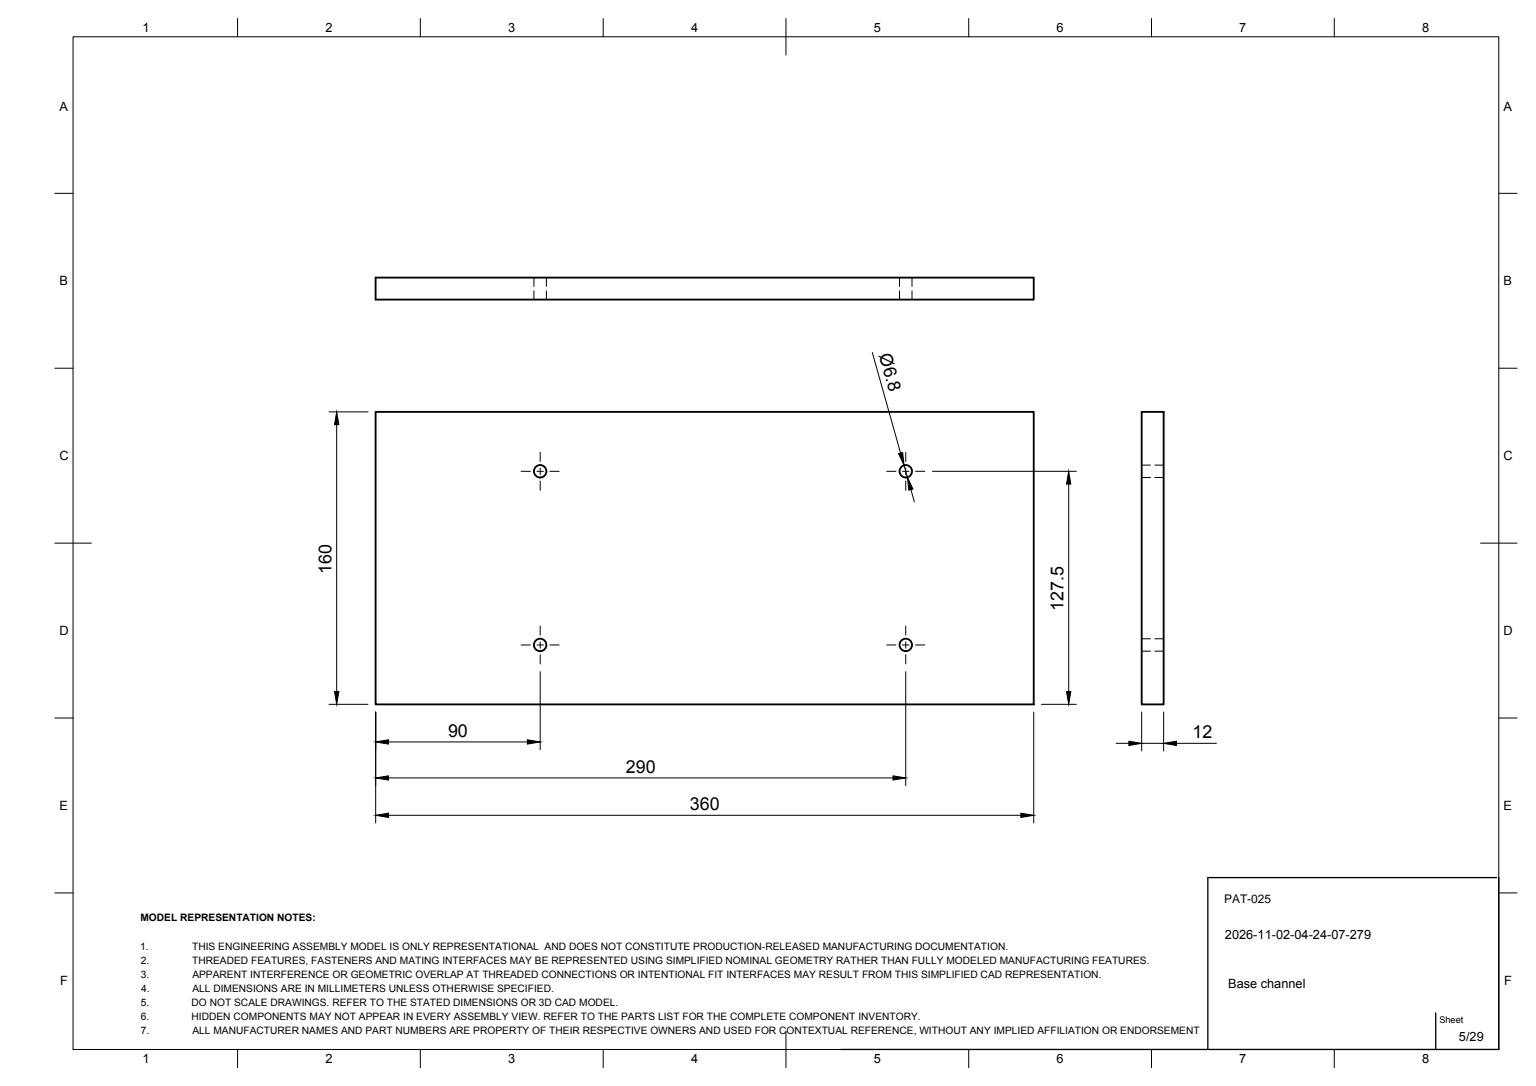
ISO-10303-21;
HEADER;
/* Generated by software containing ST-Developer
 * from STEP Tools, Inc. (www.steptools.com) 
 */

FILE_DESCRIPTION(
/* description */ ('Counter shaft with two pulleys and keyed hub'),
/* implementation_level */ '2;1');

FILE_NAME(
/* name */ 'Base channel.step',
/* time_stamp */ '2026-10-27T10:46:10-07:00',
/* author */ (''),
/* organization */ (''),
/* preprocessor_version */ 'ST-DEVELOPER v20.2',
/* originating_system */ 'Autodesk Translation Framework v15.17.0.0',
/* authorisation */ '');

FILE_SCHEMA (('AUTOMOTIVE_DESIGN { 1 0 10303 214 3 1 1 }'));
ENDSEC;

DATA;
#10=MECHANICAL_DESIGN_GEOMETRIC_PRESENTATION_REPRESENTATION('',(#290),#10821);
#240=SHAPE_REPRESENTATION_RELATIONSHIP('SRR','None',#10926,#265);
#265=ADVANCED_BREP_SHAPE_REPRESENTATION('',(#316),#10794);
#290=STYLED_ITEM('',(#11114),#316);
#316=MANIFOLD_SOLID_BREP('Body1',#5573);
#340=FACE_BOUND('',#911,.T.);
#341=FACE_BOUND('',#912,.T.);
#342=FACE_BOUND('',#913,.T.);
#343=FACE_BOUND('',#914,.T.);
#344=FACE_BOUND('',#916,.T.);
#345=FACE_BOUND('',#917,.T.);
#346=FACE_BOUND('',#918,.T.);
#347=FACE_BOUND('',#919,.T.);
#431=PLANE('',#5892);
#432=PLANE('',#5893);
#433=PLANE('',#5894);
#434=PLANE('',#5895);
#435=PLANE('',#5896);
#436=PLANE('',#5897);
#588=FACE_OUTER_BOUND('',#902,.T.);
#589=FACE_OUTER_BOUND('',#903,.T.);
#590=FACE_OUTER_BOUND('',#904,.T.);
#591=FACE_OUTER_BOUND('',#905,.T.);
#592=FACE_OUTER_BOUND('',#906,.T.);
#593=FACE_OUTER_BOUND('',#907,.T.);
#594=FACE_OUTER_BOUND('',#908,.T.);
#595=FACE_OUTER_BOUND('',#909,.T.);
#596=FACE_OUTER_BOUND('',#910,.T.);
#597=FACE_OUTER_BOUND('',#915,.T.);
#902=EDGE_LOOP('',(#3629,#3630,#3631,#3632));
#903=EDGE_LOOP('',(#3633,#3634,#3635,#3636));
#904=EDGE_LOOP('',(#3637,#3638,#3639,#3640));
#905=EDGE_LOOP('',(#3641,#3642,#3643,#3644));
#906=EDGE_LOOP('',(#3645,#3646,#3647,#3648));
#907=EDGE_LOOP('',(#3649,#3650,#3651,#3652));
#908=EDGE_LOOP('',(#3653,#3654,#3655,#3656));
#909=EDGE_LOOP('',(#3657,#3658,#3659,#3660));
#910=EDGE_LOOP('',(#3661,#3662,#3663,#3664));
#911=EDGE_LOOP('',(#3665));
#912=EDGE_LOOP('',(#3666));
#913=EDGE_LOOP('',(#3667));
#914=EDGE_LOOP('',(#3668));
#915=EDGE_LOOP('',(#3669,#3670,#3671,#3672));
#916=EDGE_LOOP('',(#3673));
#917=EDGE_LOOP('',(#3674));
#918=EDGE_LOOP('',(#3675));
#919=EDGE_LOOP('',(#3676));
#1307=LINE('',#8319,#1696);
#1308=LINE('',#8325,#1697);
#1309=LINE('',#8331,#1698);
#1310=LINE('',#8337,#1699);
#1311=LINE('',#8342,#1700);
#1312=LINE('',#8344,#1701);
#1313=LINE('',#8346,#1702);
#1314=LINE('',#8347,#1703);
#1315=LINE('',#8350,#1704);
#1316=LINE('',#8352,#1705);
#1317=LINE('',#8353,#1706);
#1318=LINE('',#8356,#1707);
#1319=LINE('',#8358,#1708);
#1320=LINE('',#8359,#1709);
#1321=LINE('',#8361,#1710);
#1322=LINE('',#8362,#1711);
#1696=VECTOR('',#6569,0.34);
#1697=VECTOR('',#6576,0.34);
#1698=VECTOR('',#6583,0.34);
#1699=VECTOR('',#6590,0.34);
#1700=VECTOR('',#6595,1.);
#1701=VECTOR('',#6596,1.);
#1702=VECTOR('',#6597,1.);
#1703=VECTOR('',#6598,1.);
#1704=VECTOR('',#6601,1.);
#1705=VECTOR('',#6602,1.);
#1706=VECTOR('',#6603,1.);
#1707=VECTOR('',#6606,1.);
#1708=VECTOR('',#6607,1.);
#1709=VECTOR('',#6608,1.);
#1710=VECTOR('',#6611,1.);
#1711=VECTOR('',#6612,1.);
#2085=CIRCLE('',#5881,0.34);
#2086=CIRCLE('',#5882,0.34);
#2087=CIRCLE('',#5884,0.34);
#2088=CIRCLE('',#5885,0.34);
#2089=CIRCLE('',#5887,0.34);
#2090=CIRCLE('',#5888,0.34);
#2091=CIRCLE('',#5890,0.34);
#2092=CIRCLE('',#5891,0.34);
#2384=VERTEX_POINT('',#8316);
#2385=VERTEX_POINT('',#8318);
#2386=VERTEX_POINT('',#8322);
#2387=VERTEX_POINT('',#8324);
#2388=VERTEX_POINT('',#8328);
#2389=VERTEX_POINT('',#8330);
#2390=VERTEX_POINT('',#8334);
#2391=VERTEX_POINT('',#8336);
#2392=VERTEX_POINT('',#8340);
#2393=VERTEX_POINT('',#8341);
#2394=VERTEX_POINT('',#8343);
#2395=VERTEX_POINT('',#8345);
#2396=VERTEX_POINT('',#8349);
#2397=VERTEX_POINT('',#8351);
#2398=VERTEX_POINT('',#8355);
#2399=VERTEX_POINT('',#8357);
#2887=EDGE_CURVE('',#2384,#2384,#2085,.T.);
#2888=EDGE_CURVE('',#2384,#2385,#1307,.T.);
#2889=EDGE_CURVE('',#2385,#2385,#2086,.T.);
#2890=EDGE_CURVE('',#2386,#2386,#2087,.T.);
#2891=EDGE_CURVE('',#2386,#2387,#1308,.T.);
#2892=EDGE_CURVE('',#2387,#2387,#2088,.T.);
#2893=EDGE_CURVE('',#2388,#2388,#2089,.T.);
#2894=EDGE_CURVE('',#2388,#2389,#1309,.T.);
#2895=EDGE_CURVE('',#2389,#2389,#2090,.T.);
#2896=EDGE_CURVE('',#2390,#2390,#2091,.T.);
#2897=EDGE_CURVE('',#2390,#2391,#1310,.T.);
#2898=EDGE_CURVE('',#2391,#2391,#2092,.T.);
#2899=EDGE_CURVE('',#2392,#2393,#1311,.T.);
#2900=EDGE_CURVE('',#2393,#2394,#1312,.T.);
#2901=EDGE_CURVE('',#2395,#2394,#1313,.T.);
#2902=EDGE_CURVE('',#2392,#2395,#1314,.T.);
#2903=EDGE_CURVE('',#2396,#2392,#1315,.T.);
#2904=EDGE_CURVE('',#2397,#2395,#1316,.T.);
#2905=EDGE_CURVE('',#2396,#2397,#1317,.T.);
#2906=EDGE_CURVE('',#2398,#2396,#1318,.T.);
#2907=EDGE_CURVE('',#2399,#2397,#1319,.T.);
#2908=EDGE_CURVE('',#2398,#2399,#1320,.T.);
#2909=EDGE_CURVE('',#2393,#2398,#1321,.T.);
#2910=EDGE_CURVE('',#2394,#2399,#1322,.T.);
#3629=ORIENTED_EDGE('',*,*,#2887,.F.);
#3630=ORIENTED_EDGE('',*,*,#2888,.T.);
#3631=ORIENTED_EDGE('',*,*,#2889,.F.);
#3632=ORIENTED_EDGE('',*,*,#2888,.F.);
#3633=ORIENTED_EDGE('',*,*,#2890,.F.);
#3634=ORIENTED_EDGE('',*,*,#2891,.T.);
#3635=ORIENTED_EDGE('',*,*,#2892,.F.);
#3636=ORIENTED_EDGE('',*,*,#2891,.F.);
#3637=ORIENTED_EDGE('',*,*,#2893,.F.);
#3638=ORIENTED_EDGE('',*,*,#2894,.T.);
#3639=ORIENTED_EDGE('',*,*,#2895,.F.);
#3640=ORIENTED_EDGE('',*,*,#2894,.F.);
#3641=ORIENTED_EDGE('',*,*,#2896,.F.);
#3642=ORIENTED_EDGE('',*,*,#2897,.T.);
#3643=ORIENTED_EDGE('',*,*,#2898,.F.);
#3644=ORIENTED_EDGE('',*,*,#2897,.F.);
#3645=ORIENTED_EDGE('',*,*,#2899,.T.);
#3646=ORIENTED_EDGE('',*,*,#2900,.T.);
#3647=ORIENTED_EDGE('',*,*,#2901,.F.);
#3648=ORIENTED_EDGE('',*,*,#2902,.F.);
#3649=ORIENTED_EDGE('',*,*,#2903,.T.);
#3650=ORIENTED_EDGE('',*,*,#2902,.T.);
#3651=ORIENTED_EDGE('',*,*,#2904,.F.);
#3652=ORIENTED_EDGE('',*,*,#2905,.F.);
#3653=ORIENTED_EDGE('',*,*,#2906,.T.);
#3654=ORIENTED_EDGE('',*,*,#2905,.T.);
#3655=ORIENTED_EDGE('',*,*,#2907,.F.);
#3656=ORIENTED_EDGE('',*,*,#2908,.F.);
#3657=ORIENTED_EDGE('',*,*,#2909,.T.);
#3658=ORIENTED_EDGE('',*,*,#2908,.T.);
#3659=ORIENTED_EDGE('',*,*,#2910,.F.);
#3660=ORIENTED_EDGE('',*,*,#2900,.F.);
#3661=ORIENTED_EDGE('',*,*,#2910,.T.);
#3662=ORIENTED_EDGE('',*,*,#2907,.T.);
#3663=ORIENTED_EDGE('',*,*,#2904,.T.);
#3664=ORIENTED_EDGE('',*,*,#2901,.T.);
#3665=ORIENTED_EDGE('',*,*,#2889,.T.);
#3666=ORIENTED_EDGE('',*,*,#2892,.T.);
#3667=ORIENTED_EDGE('',*,*,#2895,.T.);
#3668=ORIENTED_EDGE('',*,*,#2898,.T.);
#3669=ORIENTED_EDGE('',*,*,#2909,.F.);
#3670=ORIENTED_EDGE('',*,*,#2899,.F.);
#3671=ORIENTED_EDGE('',*,*,#2903,.F.);
#3672=ORIENTED_EDGE('',*,*,#2906,.F.);
#3673=ORIENTED_EDGE('',*,*,#2887,.T.);
#3674=ORIENTED_EDGE('',*,*,#2890,.T.);
#3675=ORIENTED_EDGE('',*,*,#2893,.T.);
#3676=ORIENTED_EDGE('',*,*,#2896,.T.);
#5113=CYLINDRICAL_SURFACE('',#5880,0.34);
#5114=CYLINDRICAL_SURFACE('',#5883,0.34);
#5115=CYLINDRICAL_SURFACE('',#5886,0.34);
#5116=CYLINDRICAL_SURFACE('',#5889,0.34);
#5259=ADVANCED_FACE('',(#588),#5113,.F.);
#5260=ADVANCED_FACE('',(#589),#5114,.F.);
#5261=ADVANCED_FACE('',(#590),#5115,.F.);
#5262=ADVANCED_FACE('',(#591),#5116,.F.);
#5263=ADVANCED_FACE('',(#592),#431,.T.);
#5264=ADVANCED_FACE('',(#593),#432,.T.);
#5265=ADVANCED_FACE('',(#594),#433,.T.);
#5266=ADVANCED_FACE('',(#595),#434,.T.);
#5267=ADVANCED_FACE('',(#596,#340,#341,#342,#343),#435,.T.);
#5268=ADVANCED_FACE('',(#597,#344,#345,#346,#347),#436,.F.);
#5573=CLOSED_SHELL('',(#5259,#5260,#5261,#5262,#5263,#5264,#5265,#5266,
#5267,#5268));
#5879=AXIS2_PLACEMENT_3D('',#8314,#6563,#6564);
#5880=AXIS2_PLACEMENT_3D('',#8315,#6565,#6566);
#5881=AXIS2_PLACEMENT_3D('',#8317,#6567,#6568);
#5882=AXIS2_PLACEMENT_3D('',#8320,#6570,#6571);
#5883=AXIS2_PLACEMENT_3D('',#8321,#6572,#6573);
#5884=AXIS2_PLACEMENT_3D('',#8323,#6574,#6575);
#5885=AXIS2_PLACEMENT_3D('',#8326,#6577,#6578);
#5886=AXIS2_PLACEMENT_3D('',#8327,#6579,#6580);
#5887=AXIS2_PLACEMENT_3D('',#8329,#6581,#6582);
#5888=AXIS2_PLACEMENT_3D('',#8332,#6584,#6585);
#5889=AXIS2_PLACEMENT_3D('',#8333,#6586,#6587);
#5890=AXIS2_PLACEMENT_3D('',#8335,#6588,#6589);
#5891=AXIS2_PLACEMENT_3D('',#8338,#6591,#6592);
#5892=AXIS2_PLACEMENT_3D('',#8339,#6593,#6594);
#5893=AXIS2_PLACEMENT_3D('',#8348,#6599,#6600);
#5894=AXIS2_PLACEMENT_3D('',#8354,#6604,#6605);
#5895=AXIS2_PLACEMENT_3D('',#8360,#6609,#6610);
#5896=AXIS2_PLACEMENT_3D('',#8363,#6613,#6614);
#5897=AXIS2_PLACEMENT_3D('',#8364,#6615,#6616);
#6563=DIRECTION('axis',(0.,0.,1.));
#6564=DIRECTION('refdir',(1.,0.,0.));
#6565=DIRECTION('center_axis',(0.,0.,1.));
#6566=DIRECTION('ref_axis',(1.,0.,0.));
#6567=DIRECTION('center_axis',(0.,0.,1.));
#6568=DIRECTION('ref_axis',(1.,0.,0.));
#6569=DIRECTION('',(0.,0.,1.));
#6570=DIRECTION('center_axis',(0.,0.,-1.));
#6571=DIRECTION('ref_axis',(1.,0.,0.));
#6572=DIRECTION('center_axis',(0.,0.,1.));
#6573=DIRECTION('ref_axis',(1.,0.,0.));
#6574=DIRECTION('center_axis',(0.,0.,1.));
#6575=DIRECTION('ref_axis',(1.,0.,0.));
#6576=DIRECTION('',(0.,0.,1.));
#6577=DIRECTION('center_axis',(0.,0.,-1.));
#6578=DIRECTION('ref_axis',(1.,0.,0.));
#6579=DIRECTION('center_axis',(0.,0.,1.));
#6580=DIRECTION('ref_axis',(1.,0.,0.));
#6581=DIRECTION('center_axis',(0.,0.,1.));
#6582=DIRECTION('ref_axis',(1.,0.,0.));
#6583=DIRECTION('',(0.,0.,1.));
#6584=DIRECTION('center_axis',(0.,0.,-1.));
#6585=DIRECTION('ref_axis',(1.,0.,0.));
#6586=DIRECTION('center_axis',(0.,0.,1.));
#6587=DIRECTION('ref_axis',(1.,0.,0.));
#6588=DIRECTION('center_axis',(0.,0.,1.));
#6589=DIRECTION('ref_axis',(1.,0.,0.));
#6590=DIRECTION('',(0.,0.,1.));
#6591=DIRECTION('center_axis',(0.,0.,-1.));
#6592=DIRECTION('ref_axis',(1.,0.,0.));
#6593=DIRECTION('center_axis',(0.,1.,0.));
#6594=DIRECTION('ref_axis',(-1.,0.,0.));
#6595=DIRECTION('',(-1.,0.,0.));
#6596=DIRECTION('',(0.,0.,1.));
#6597=DIRECTION('',(-1.,0.,0.));
#6598=DIRECTION('',(0.,0.,1.));
#6599=DIRECTION('center_axis',(1.,0.,0.));
#6600=DIRECTION('ref_axis',(0.,1.,0.));
#6601=DIRECTION('',(0.,1.,0.));
#6602=DIRECTION('',(0.,1.,0.));
#6603=DIRECTION('',(0.,0.,1.));
#6604=DIRECTION('center_axis',(0.,-1.,0.));
#6605=DIRECTION('ref_axis',(1.,0.,0.));
#6606=DIRECTION('',(1.,0.,0.));
#6607=DIRECTION('',(1.,0.,0.));
#6608=DIRECTION('',(0.,0.,1.));
#6609=DIRECTION('center_axis',(-1.,0.,0.));
#6610=DIRECTION('ref_axis',(0.,-1.,0.));
#6611=DIRECTION('',(0.,-1.,0.));
#6612=DIRECTION('',(0.,-1.,0.));
#6613=DIRECTION('center_axis',(0.,0.,1.));
#6614=DIRECTION('ref_axis',(1.,0.,0.));
#6615=DIRECTION('center_axis',(0.,0.,1.));
#6616=DIRECTION('ref_axis',(1.,0.,0.));
#8314=CARTESIAN_POINT('',(0.,0.,0.));
#8315=CARTESIAN_POINT('Origin',(4.75,0.,-0.1));
#8316=CARTESIAN_POINT('',(4.41,-4.163799117101E-17,0.));
#8317=CARTESIAN_POINT('Origin',(4.75,0.,0.));
#8318=CARTESIAN_POINT('',(4.41,4.163799117101E-17,1.2));
#8319=CARTESIAN_POINT('',(4.41,-4.163799117101E-17,-0.1));
#8320=CARTESIAN_POINT('Origin',(4.75,0.,1.2));
#8321=CARTESIAN_POINT('Origin',(-4.75,20.,-0.1));
#8322=CARTESIAN_POINT('',(-5.09,20.,0.));
#8323=CARTESIAN_POINT('Origin',(-4.75,20.,0.));
#8324=CARTESIAN_POINT('',(-5.09,20.,1.2));
#8325=CARTESIAN_POINT('',(-5.09,20.,-0.1));
#8326=CARTESIAN_POINT('Origin',(-4.75,20.,1.2));
#8327=CARTESIAN_POINT('Origin',(-4.75,0.,-0.1));
#8328=CARTESIAN_POINT('',(-5.09,-4.163799117101E-17,0.));
#8329=CARTESIAN_POINT('Origin',(-4.75,0.,0.));
#8330=CARTESIAN_POINT('',(-5.09,4.163799117101E-17,1.2));
#8331=CARTESIAN_POINT('',(-5.09,-4.163799117101E-17,-0.1));
#8332=CARTESIAN_POINT('Origin',(-4.75,0.,1.2));
#8333=CARTESIAN_POINT('Origin',(4.75,20.,-0.1));
#8334=CARTESIAN_POINT('',(4.41,20.,0.));
#8335=CARTESIAN_POINT('Origin',(4.75,20.,0.));
#8336=CARTESIAN_POINT('',(4.41,20.,1.2));
#8337=CARTESIAN_POINT('',(4.41,20.,-0.1));
#8338=CARTESIAN_POINT('Origin',(4.75,20.,1.2));
#8339=CARTESIAN_POINT('Origin',(8.,29.,0.));
#8340=CARTESIAN_POINT('',(8.,29.,0.));
#8341=CARTESIAN_POINT('',(-8.,29.,0.));
#8342=CARTESIAN_POINT('',(8.,29.,0.));
#8343=CARTESIAN_POINT('',(-8.,29.,1.2));
#8344=CARTESIAN_POINT('',(-8.,29.,0.));
#8345=CARTESIAN_POINT('',(8.,29.,1.2));
#8346=CARTESIAN_POINT('',(8.,29.,1.2));
#8347=CARTESIAN_POINT('',(8.,29.,0.));
#8348=CARTESIAN_POINT('Origin',(8.,-7.,0.));
#8349=CARTESIAN_POINT('',(8.,-7.,0.));
#8350=CARTESIAN_POINT('',(8.,-7.,0.));
#8351=CARTESIAN_POINT('',(8.,-7.,1.2));
#8352=CARTESIAN_POINT('',(8.,-7.,1.2));
#8353=CARTESIAN_POINT('',(8.,-7.,0.));
#8354=CARTESIAN_POINT('Origin',(-8.,-7.,0.));
#8355=CARTESIAN_POINT('',(-8.,-7.,0.));
#8356=CARTESIAN_POINT('',(-8.,-7.,0.));
#8357=CARTESIAN_POINT('',(-8.,-7.,1.2));
#8358=CARTESIAN_POINT('',(-8.,-7.,1.2));
#8359=CARTESIAN_POINT('',(-8.,-7.,0.));
#8360=CARTESIAN_POINT('Origin',(-8.,29.,0.));
#8361=CARTESIAN_POINT('',(-8.,29.,0.));
#8362=CARTESIAN_POINT('',(-8.,29.,1.2));
#8363=CARTESIAN_POINT('Origin',(0.,11.,1.2));
#8364=CARTESIAN_POINT('Origin',(0.,11.,0.));
#10764=UNCERTAINTY_MEASURE_WITH_UNIT(LENGTH_MEASURE(0.001),#10822,
'DISTANCE_ACCURACY_VALUE',
'Maximum model space distance between geometric entities at asserted c
onnectivities');
#10791=UNCERTAINTY_MEASURE_WITH_UNIT(LENGTH_MEASURE(0.001),#10822,
'DISTANCE_ACCURACY_VALUE',
'Maximum model space distance between geometric entities at asserted c
onnectivities');
#10794=(
GEOMETRIC_REPRESENTATION_CONTEXT(3)
GLOBAL_UNCERTAINTY_ASSIGNED_CONTEXT((#10764))
GLOBAL_UNIT_ASSIGNED_CONTEXT((#10822,#10824,#10825))
REPRESENTATION_CONTEXT('','3D')
);
#10821=(
GEOMETRIC_REPRESENTATION_CONTEXT(3)
GLOBAL_UNCERTAINTY_ASSIGNED_CONTEXT((#10791))
GLOBAL_UNIT_ASSIGNED_CONTEXT((#10822,#10824,#10825))
REPRESENTATION_CONTEXT('','3D')
);
#10822=(
LENGTH_UNIT()
NAMED_UNIT(*)
SI_UNIT(.CENTI.,.METRE.)
);
#10824=(
NAMED_UNIT(*)
PLANE_ANGLE_UNIT()
SI_UNIT($,.RADIAN.)
);
#10825=(
NAMED_UNIT(*)
SI_UNIT($,.STERADIAN.)
SOLID_ANGLE_UNIT()
);
#10828=SHAPE_DEFINITION_REPRESENTATION(#10857,#10926);
#10857=PRODUCT_DEFINITION_SHAPE('',$,#10956);
#10926=SHAPE_REPRESENTATION('',(#5879),#10794);
#10953=PRODUCT_DEFINITION_CONTEXT('part definition',#11042,'design');
#10956=PRODUCT_DEFINITION('Base channel','Base channel',#10985,#10953);
#10985=PRODUCT_DEFINITION_FORMATION('',$,#11046);
#11042=APPLICATION_CONTEXT(
'Core Data for Automotive Mechanical Design Process');
#11043=PRODUCT_CONTEXT('part definition',#11042,'mechanical');
#11046=PRODUCT('Base channel','Base channel','Base channel',(#11043));
#11108=COLOUR_RGB('Dark Blue',0.08,0.2,0.34);
#11109=FILL_AREA_STYLE_COLOUR('',#11108);
#11110=FILL_AREA_STYLE('',(#11109));
#11111=SURFACE_STYLE_FILL_AREA(#11110);
#11112=SURFACE_SIDE_STYLE('',(#11111));
#11113=SURFACE_STYLE_USAGE(.BOTH.,#11112);
#11114=PRESENTATION_STYLE_ASSIGNMENT((#11113));
ENDSEC;
END-ISO-10303-21;
